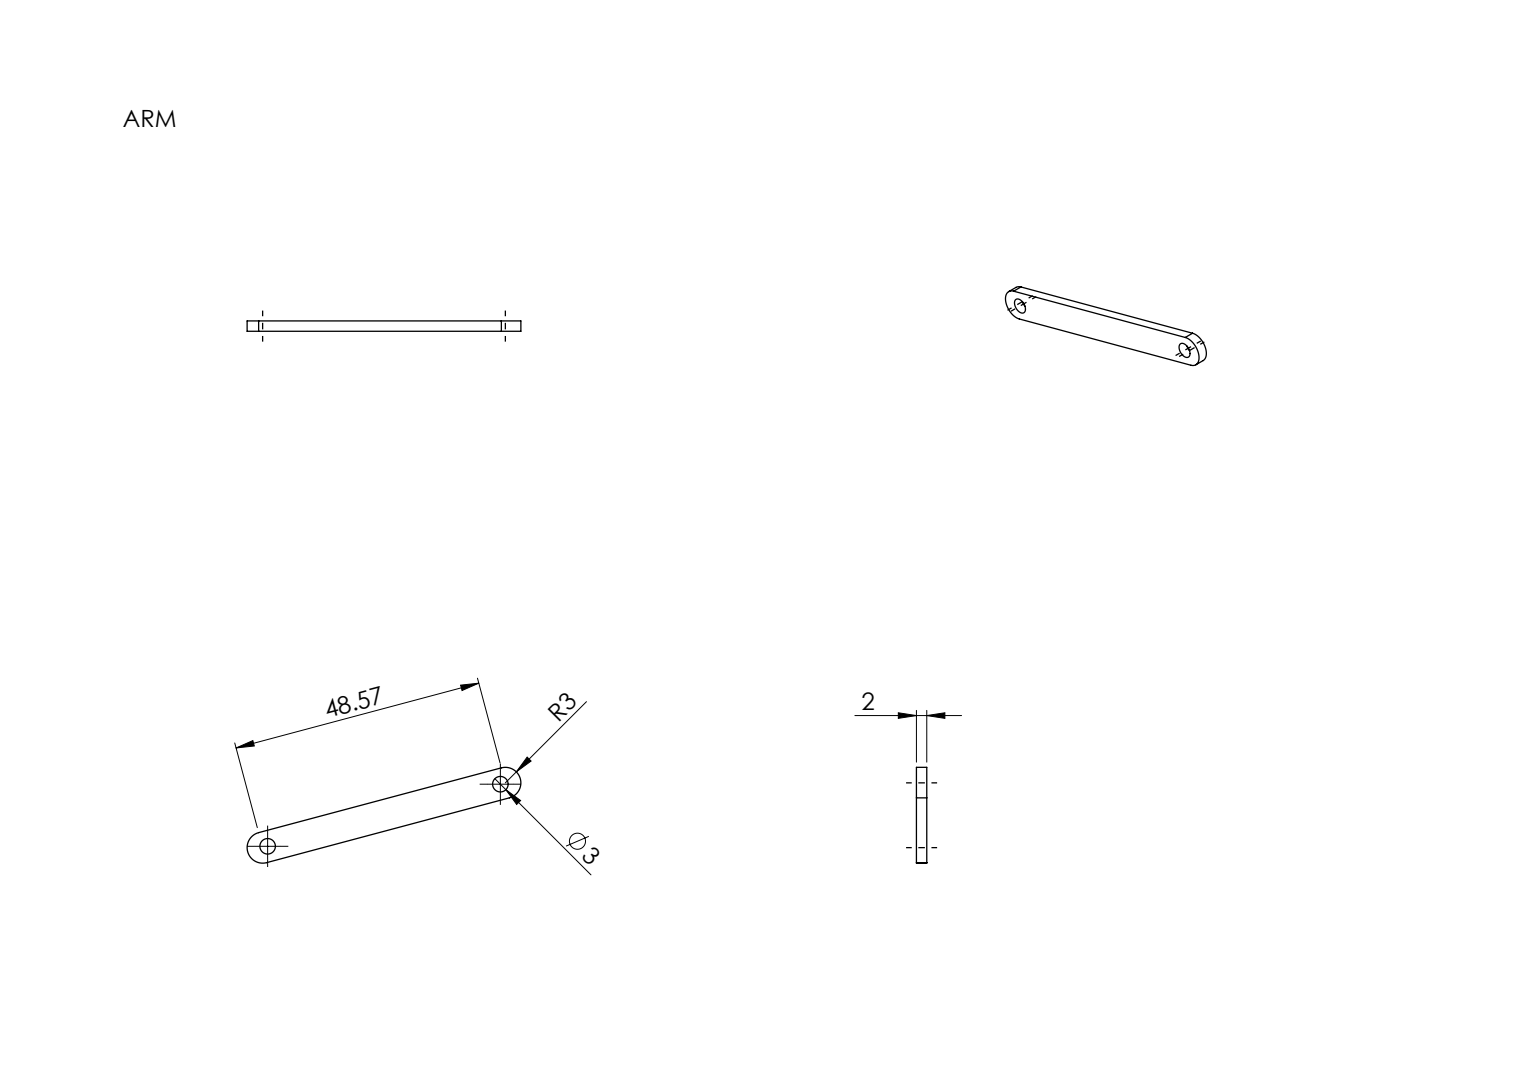
ISO-10303-21;
HEADER;
FILE_DESCRIPTION (('STEP AP214'),
    '1' );
FILE_NAME ('arm.step',
    '2026-10-04T07:56:41',
    ( '' ),
    ( '' ),
    'SwSTEP 2.0',
    'SolidWorks 2026',
    '' );
FILE_SCHEMA (( 'AUTOMOTIVE_DESIGN' ));
ENDSEC;

DATA;
#19=LINE ( 'NONE', #2774, #674 ) ;
#51=CIRCLE ( 'NONE', #1949, 3.000000000000000000 ) ;
#101=CARTESIAN_POINT ( 'NONE',  ( 46.73922289128223895, -17.64104216824340199, 4.500000000000000888 ) ) ;
#128=FACE_OUTER_BOUND ( 'NONE', #7423, .T. ) ;
#133=FACE_OUTER_BOUND ( 'NONE', #6862, .T. ) ;
#143=ORIENTED_EDGE ( 'NONE', *, *, #1238, .T. ) ;
#163=EDGE_LOOP ( 'NONE', ( #6818, #3032, #7905, #4249 ) ) ;
#171=FACE_OUTER_BOUND ( 'NONE', #565, .T. ) ;
#212=CARTESIAN_POINT ( 'NONE',  ( -0.9662349396012467340, -27.25766265056033433, 4.500000000000000888 ) ) ;
#225=SURFACE_STYLE_FILL_AREA ( #2174 ) ;
#261=CARTESIAN_POINT ( 'NONE',  ( 46.73922289128223895, -17.64104216824340199, 4.500000000000000888 ) ) ;
#270=DIRECTION ( 'NONE',  ( -0.000000000000000000, -0.000000000000000000, -1.000000000000000000 ) ) ;
#273=DIRECTION ( 'NONE',  ( 0.000000000000000000, 0.000000000000000000, 1.000000000000000000 ) ) ;
#277=ADVANCED_FACE ( 'NONE', ( #133 ), #3970, .F. ) ;
#318=LINE ( 'NONE', #2975, #6253 ) ;
#332=ORIENTED_EDGE ( 'NONE', *, *, #7144, .F. ) ;
#384=DIRECTION ( 'NONE',  ( -1.000000000000000000, 0.000000000000000000, 0.000000000000000000 ) ) ;
#386=AXIS2_PLACEMENT_3D ( 'NONE', #1428, #3953, #5087 ) ;
#402=CARTESIAN_POINT ( 'NONE',  ( 0.7729879516809982087, -29.89870481880373987, 4.500000000000000888 ) ) ;
#425=VERTEX_POINT ( 'NONE', #5144 ) ;
#426=CARTESIAN_POINT ( 'NONE',  ( 45.96623493960122886, -14.74233734943963192, 2.500000000000000888 ) ) ;
#468=( NAMED_UNIT ( * ) PLANE_ANGLE_UNIT ( ) SI_UNIT ( $, .RADIAN. ) );
#504=FACE_OUTER_BOUND ( 'NONE', #5035, .T. ) ;
#521=AXIS2_PLACEMENT_3D ( 'NONE', #5224, #627, #804 ) ;
#540=VERTEX_POINT ( 'NONE', #5837 ) ;
#565=EDGE_LOOP ( 'NONE', ( #768, #2129, #3059, #5475 ) ) ;
#577=VERTEX_POINT ( 'NONE', #7832 ) ;
#602=EDGE_CURVE ( 'NONE', #5645, #577, #5831, .T. ) ;
#627=DIRECTION ( 'NONE',  ( -0.000000000000000000, -0.000000000000000000, -1.000000000000000000 ) ) ;
#672=( GEOMETRIC_REPRESENTATION_CONTEXT ( 3 ) GLOBAL_UNCERTAINTY_ASSIGNED_CONTEXT ( ( #2169 ) ) GLOBAL_UNIT_ASSIGNED_CONTEXT ( ( #902, #4727, #5913 ) ) REPRESENTATION_CONTEXT ( 'NONE', 'WORKASPACE' ) );
#673=FACE_OUTER_BOUND ( 'NONE', #163, .T. ) ;
#674=VECTOR ( 'NONE', #2142, 1000.000000000000000 ) ;
#693=DIRECTION ( 'NONE',  ( 0.000000000000000000, 0.000000000000000000, 1.000000000000000000 ) ) ;
#705=ORIENTED_EDGE ( 'NONE', *, *, #1358, .T. ) ;
#729=CIRCLE ( 'NONE', #4630, 1.500000000000001998 ) ;
#768=ORIENTED_EDGE ( 'NONE', *, *, #6942, .T. ) ;
#772=( LENGTH_UNIT ( ) NAMED_UNIT ( * ) SI_UNIT ( .MILLI., .METRE. ) );
#777=EDGE_CURVE ( 'NONE', #3733, #7693, #19, .T. ) ;
#804=DIRECTION ( 'NONE',  ( -1.000000000000000000, 0.000000000000000000, 0.000000000000000000 ) ) ;
#805=CIRCLE ( 'NONE', #4298, 3.000000000000000000 ) ;
#816=EDGE_LOOP ( 'NONE', ( #5885, #8217, #3994, #3810 ) ) ;
#862=VECTOR ( 'NONE', #1618, 1000.000000000000227 ) ;
#902=( LENGTH_UNIT ( ) NAMED_UNIT ( * ) SI_UNIT ( .MILLI., .METRE. ) );
#937=EDGE_CURVE ( 'NONE', #8122, #5636, #7138, .T. ) ;
#944=VECTOR ( 'NONE', #2202, 1000.000000000000000 ) ;
#971=DIRECTION ( 'NONE',  ( -1.000000000000000000, 0.000000000000000000, 0.000000000000000000 ) ) ;
#980=CYLINDRICAL_SURFACE ( 'NONE', #1948, 1.499999999999994449 ) ;
#998=CIRCLE ( 'NONE', #3155, 1.500000000000001998 ) ;
#1037=ADVANCED_FACE ( 'NONE', ( #3889 ), #7135, .F. ) ;
#1053=DIRECTION ( 'NONE',  ( 0.000000000000000000, 0.000000000000000000, 1.000000000000000000 ) ) ;
#1078=CARTESIAN_POINT ( 'NONE',  ( 6.123233995736760366E-16, -27.00000000000000000, 4.500000000000000888 ) ) ;
#1102=FILL_AREA_STYLE ('',( #6916 ) ) ;
#1137=CARTESIAN_POINT ( 'NONE',  ( 45.96623493960122886, -14.74233734943963192, 4.500000000000000888 ) ) ;
#1238=EDGE_CURVE ( 'NONE', #3733, #5980, #6033, .T. ) ;
#1256=AXIS2_PLACEMENT_3D ( 'NONE', #1926, #3778, #2010 ) ;
#1265=( GEOMETRIC_REPRESENTATION_CONTEXT ( 3 ) GLOBAL_UNCERTAINTY_ASSIGNED_CONTEXT ( ( #3607 ) ) GLOBAL_UNIT_ASSIGNED_CONTEXT ( ( #7000, #468, #5646 ) ) REPRESENTATION_CONTEXT ( 'NONE', 'WORKASPACE' ) );
#1283=DIRECTION ( 'NONE',  ( 0.000000000000000000, 0.000000000000000000, 1.000000000000000000 ) ) ;
#1345=ORIENTED_EDGE ( 'NONE', *, *, #2125, .T. ) ;
#1358=EDGE_CURVE ( 'NONE', #8122, #577, #2207, .T. ) ;
#1392=PRODUCT_DEFINITION ( 'UNKNOWN', '', #2424, #5360 ) ;
#1394=PLANE ( 'NONE',  #6055 ) ;
#1402=DIRECTION ( 'NONE',  ( -1.000000000000000000, 0.000000000000000000, 0.000000000000000000 ) ) ;
#1428=CARTESIAN_POINT ( 'NONE',  ( 45.00000000000000000, -14.99999999999999467, 2.500000000000000888 ) ) ;
#1470=DIRECTION ( 'NONE',  ( -0.000000000000000000, -0.000000000000000000, -1.000000000000000000 ) ) ;
#1472=ORIENTED_EDGE ( 'NONE', *, *, #5256, .T. ) ;
#1493=( NAMED_UNIT ( * ) PLANE_ANGLE_UNIT ( ) SI_UNIT ( $, .RADIAN. ) );
#1536=VECTOR ( 'NONE', #1470, 1000.000000000000000 ) ;
#1541=CARTESIAN_POINT ( 'NONE',  ( 45.00000000000000000, -14.99999999999999467, 4.500000000000000888 ) ) ;
#1545=EDGE_CURVE ( 'NONE', #2326, #3416, #2265, .T. ) ;
#1594=VERTEX_POINT ( 'NONE', #6433 ) ;
#1605=CARTESIAN_POINT ( 'NONE',  ( 45.96623493960122886, -14.74233734943963192, 4.500000000000000888 ) ) ;
#1618=DIRECTION ( 'NONE',  ( 0.9662349396012460678, 0.2576626505603330508, -0.000000000000000000 ) ) ;
#1654=CARTESIAN_POINT ( 'NONE',  ( 45.19324698792023298, -11.84363253063589205, 4.500000000000000888 ) ) ;
#1674=AXIS2_PLACEMENT_3D ( 'NONE', #2882, #3591, #384 ) ;
#1728=VECTOR ( 'NONE', #6153, 1000.000000000000000 ) ;
#1731=ORIENTED_EDGE ( 'NONE', *, *, #2146, .T. ) ;
#1756=DIRECTION ( 'NONE',  ( 1.000000000000000000, 0.000000000000000000, 0.000000000000000000 ) ) ;
#1782=ORIENTED_EDGE ( 'NONE', *, *, #937, .T. ) ;
#1813=MECHANICAL_DESIGN_GEOMETRIC_PRESENTATION_REPRESENTATION('',(#6914),#1265);
#1818=CIRCLE ( 'NONE', #2086, 1.499999999999994449 ) ;
#1882=ORIENTED_EDGE ( 'NONE', *, *, #4850, .T. ) ;
#1926=CARTESIAN_POINT ( 'NONE',  ( -0.9662349396012467340, -27.25766265056033433, 2.500000000000000888 ) ) ;
#1933=SHAPE_REPRESENTATION ( 'arm', ( #2840 ), #5779 ) ;
#1946=EDGE_CURVE ( 'NONE', #1594, #540, #729, .T. ) ;
#1948=AXIS2_PLACEMENT_3D ( 'NONE', #4723, #2211, #6078 ) ;
#1949=AXIS2_PLACEMENT_3D ( 'NONE', #4301, #7678, #4461 ) ;
#1954=FACE_BOUND ( 'NONE', #3515, .T. ) ;
#1994=DIRECTION ( 'NONE',  ( 0.000000000000000000, 0.000000000000000000, 1.000000000000000000 ) ) ;
#2008=CARTESIAN_POINT ( 'NONE',  ( 45.00000000000000000, -14.99999999999999467, 4.500000000000000888 ) ) ;
#2010=DIRECTION ( 'NONE',  ( -1.000000000000000000, 0.000000000000000000, 0.000000000000000000 ) ) ;
#2016=CARTESIAN_POINT ( 'NONE',  ( 45.00000000000000000, -14.99999999999999467, 2.500000000000000888 ) ) ;
#2038=CARTESIAN_POINT ( 'NONE',  ( 6.123233995736760366E-16, -27.00000000000000000, 2.500000000000000888 ) ) ;
#2050=FILL_AREA_STYLE_COLOUR ( '', #3641 ) ;
#2077=CARTESIAN_POINT ( 'NONE',  ( 0.7729879516809982087, -29.89870481880373987, 4.500000000000000888 ) ) ;
#2086=AXIS2_PLACEMENT_3D ( 'NONE', #2008, #1283, #2469 ) ;
#2093=ORIENTED_EDGE ( 'NONE', *, *, #2146, .F. ) ;
#2111=ORIENTED_EDGE ( 'NONE', *, *, #6840, .F. ) ;
#2117=EDGE_CURVE ( 'NONE', #425, #6564, #6175, .T. ) ;
#2125=EDGE_CURVE ( 'NONE', #540, #2326, #318, .T. ) ;
#2129=ORIENTED_EDGE ( 'NONE', *, *, #7263, .F. ) ;
#2142=DIRECTION ( 'NONE',  ( -0.9662349396012451797, -0.2576626505603366590, -0.000000000000000000 ) ) ;
#2146=EDGE_CURVE ( 'NONE', #5636, #8122, #1818, .T. ) ;
#2149=CIRCLE ( 'NONE', #386, 1.499999999999994449 ) ;
#2169=UNCERTAINTY_MEASURE_WITH_UNIT (LENGTH_MEASURE( 1.000000000000000082E-05 ), #902, 'distance_accuracy_value', 'NONE');
#2174=FILL_AREA_STYLE ('',( #2050 ) ) ;
#2202=DIRECTION ( 'NONE',  ( -0.000000000000000000, -0.000000000000000000, -1.000000000000000000 ) ) ;
#2207=LINE ( 'NONE', #4719, #1728 ) ;
#2211=DIRECTION ( 'NONE',  ( -0.000000000000000000, -0.000000000000000000, -1.000000000000000000 ) ) ;
#2228=ORIENTED_EDGE ( 'NONE', *, *, #1545, .T. ) ;
#2246=FACE_OUTER_BOUND ( 'NONE', #816, .T. ) ;
#2255=ORIENTED_EDGE ( 'NONE', *, *, #937, .F. ) ;
#2265=CIRCLE ( 'NONE', #8315, 1.500000000000001998 ) ;
#2310=ORIENTED_EDGE ( 'NONE', *, *, #602, .F. ) ;
#2312=EDGE_LOOP ( 'NONE', ( #2228, #1882 ) ) ;
#2326=VERTEX_POINT ( 'NONE', #5199 ) ;
#2327=DIRECTION ( 'NONE',  ( 0.000000000000000000, 0.000000000000000000, 1.000000000000000000 ) ) ;
#2335=CARTESIAN_POINT ( 'NONE',  ( 0.7729879516809982087, -29.89870481880373987, 2.500000000000000888 ) ) ;
#2385=DIRECTION ( 'NONE',  ( 0.000000000000000000, 0.000000000000000000, 1.000000000000000000 ) ) ;
#2424=PRODUCT_DEFINITION_FORMATION_WITH_SPECIFIED_SOURCE ( 'ANY', '', #3664, .NOT_KNOWN. ) ;
#2469=DIRECTION ( 'NONE',  ( 1.000000000000000000, 0.000000000000000000, 0.000000000000000000 ) ) ;
#2475=CIRCLE ( 'NONE', #7188, 3.000000000000002665 ) ;
#2556=DIRECTION ( 'NONE',  ( -0.000000000000000000, -0.000000000000000000, -1.000000000000000000 ) ) ;
#2594=ADVANCED_FACE ( 'NONE', ( #4778 ), #2726, .T. ) ;
#2625=DIRECTION ( 'NONE',  ( 0.000000000000000000, 0.000000000000000000, 1.000000000000000000 ) ) ;
#2635=CLOSED_SHELL ( 'NONE', ( #1037, #4519, #4754, #4844, #6356, #7819, #6759, #2594, #7467, #277, #4433 ) ) ;
#2699=CARTESIAN_POINT ( 'NONE',  ( 46.49999999999999289, -14.99999999999999467, 2.500000000000000888 ) ) ;
#2715=CARTESIAN_POINT ( 'NONE',  ( 6.123233995736760366E-16, -27.00000000000000000, 4.500000000000000888 ) ) ;
#2726=CYLINDRICAL_SURFACE ( 'NONE', #4756, 3.000000000000000000 ) ;
#2729=EDGE_CURVE ( 'NONE', #7693, #2822, #6003, .T. ) ;
#2755=VECTOR ( 'NONE', #2556, 1000.000000000000000 ) ;
#2774=CARTESIAN_POINT ( 'NONE',  ( 44.22701204831900412, -12.10129518119625658, 4.500000000000000888 ) ) ;
#2804=ORIENTED_EDGE ( 'NONE', *, *, #602, .T. ) ;
#2812=ORIENTED_EDGE ( 'NONE', *, *, #5575, .F. ) ;
#2822=VERTEX_POINT ( 'NONE', #7439 ) ;
#2840=AXIS2_PLACEMENT_3D ( 'NONE', #8120, #5497, #1756 ) ;
#2877=LINE ( 'NONE', #6702, #6242 ) ;
#2882=CARTESIAN_POINT ( 'NONE',  ( -0.9662349396012467340, -27.25766265056033433, 4.500000000000000888 ) ) ;
#2963=DIRECTION ( 'NONE',  ( 0.000000000000000000, 0.000000000000000000, 1.000000000000000000 ) ) ;
#2975=CARTESIAN_POINT ( 'NONE',  ( -1.500000000000001332, -27.00000000000000000, 4.500000000000000888 ) ) ;
#2994=DIRECTION ( 'NONE',  ( 0.000000000000000000, 0.000000000000000000, 1.000000000000000000 ) ) ;
#3011=EDGE_CURVE ( 'NONE', #540, #1594, #998, .T. ) ;
#3032=ORIENTED_EDGE ( 'NONE', *, *, #4118, .T. ) ;
#3041=DIRECTION ( 'NONE',  ( -0.000000000000000000, -0.000000000000000000, -1.000000000000000000 ) ) ;
#3055=EDGE_LOOP ( 'NONE', ( #2111, #7565, #4948, #332, #7058 ) ) ;
#3059=ORIENTED_EDGE ( 'NONE', *, *, #2117, .F. ) ;
#3102=STYLED_ITEM ( 'NONE', ( #3979 ), #4379 ) ;
#3103=ORIENTED_EDGE ( 'NONE', *, *, #2125, .F. ) ;
#3104=CARTESIAN_POINT ( 'NONE',  ( 45.96623493960122886, -14.74233734943963192, 2.500000000000000888 ) ) ;
#3138=ORIENTED_EDGE ( 'NONE', *, *, #6646, .T. ) ;
#3155=AXIS2_PLACEMENT_3D ( 'NONE', #6255, #2385, #3645 ) ;
#3160=LINE ( 'NONE', #3790, #3546 ) ;
#3161=VECTOR ( 'NONE', #3731, 1000.000000000000114 ) ;
#3183=ORIENTED_EDGE ( 'NONE', *, *, #1946, .T. ) ;
#3295=AXIS2_PLACEMENT_3D ( 'NONE', #2016, #693, #6600 ) ;
#3296=COLOUR_RGB ( '', 0.66274510, 0.83137255, 0.94901961) ;
#3370=AXIS2_PLACEMENT_3D ( 'NONE', #1605, #4170, #971 ) ;
#3416=VERTEX_POINT ( 'NONE', #5319 ) ;
#3471=ORIENTED_EDGE ( 'NONE', *, *, #1545, .F. ) ;
#3515=EDGE_LOOP ( 'NONE', ( #4016, #3980 ) ) ;
#3521=DIRECTION ( 'NONE',  ( 1.000000000000000000, 0.000000000000000000, 0.000000000000000000 ) ) ;
#3525=ORIENTED_EDGE ( 'NONE', *, *, #2729, .F. ) ;
#3546=VECTOR ( 'NONE', #6361, 1000.000000000000000 ) ;
#3563=ORIENTED_EDGE ( 'NONE', *, *, #7749, .F. ) ;
#3581=ORIENTED_EDGE ( 'NONE', *, *, #7144, .T. ) ;
#3591=DIRECTION ( 'NONE',  ( 0.000000000000000000, 0.000000000000000000, 1.000000000000000000 ) ) ;
#3607=UNCERTAINTY_MEASURE_WITH_UNIT (LENGTH_MEASURE( 1.000000000000000082E-05 ), #7000, 'distance_accuracy_value', 'NONE');
#3641=COLOUR_RGB ( '', 0.66274510, 0.83137255, 0.94901961) ;
#3645=DIRECTION ( 'NONE',  ( 1.000000000000000000, 0.000000000000000000, 0.000000000000000000 ) ) ;
#3664=PRODUCT ( 'arm', 'arm', '', ( #5516 ) ) ;
#3731=DIRECTION ( 'NONE',  ( 0.9662349396012461789, 0.2576626505603324402, 0.000000000000000000 ) ) ;
#3733=VERTEX_POINT ( 'NONE', #1654 ) ;
#3734=FACE_BOUND ( 'NONE', #2312, .T. ) ;
#3773=EDGE_CURVE ( 'NONE', #5980, #2822, #2877, .T. ) ;
#3775=MECHANICAL_DESIGN_GEOMETRIC_PRESENTATION_REPRESENTATION('',(#3102),#672);
#3778=DIRECTION ( 'NONE',  ( 0.000000000000000000, 0.000000000000000000, 1.000000000000000000 ) ) ;
#3790=CARTESIAN_POINT ( 'NONE',  ( -3.966234939601246623, -27.25766265056033433, 4.500000000000000888 ) ) ;
#3810=ORIENTED_EDGE ( 'NONE', *, *, #7263, .T. ) ;
#3876=AXIS2_PLACEMENT_3D ( 'NONE', #7856, #7176, #1402 ) ;
#3889=FACE_OUTER_BOUND ( 'NONE', #7158, .T. ) ;
#3952=VERTEX_POINT ( 'NONE', #6989 ) ;
#3953=DIRECTION ( 'NONE',  ( 0.000000000000000000, 0.000000000000000000, 1.000000000000000000 ) ) ;
#3970=CYLINDRICAL_SURFACE ( 'NONE', #4962, 1.500000000000001998 ) ;
#3979=PRESENTATION_STYLE_ASSIGNMENT (( #5325 ) ) ;
#3980=ORIENTED_EDGE ( 'NONE', *, *, #1946, .F. ) ;
#3982=DIRECTION ( 'NONE',  ( -0.000000000000000000, -0.000000000000000000, -1.000000000000000000 ) ) ;
#3994=ORIENTED_EDGE ( 'NONE', *, *, #5256, .F. ) ;
#4016=ORIENTED_EDGE ( 'NONE', *, *, #3011, .F. ) ;
#4118=EDGE_CURVE ( 'NONE', #5910, #8028, #3160, .T. ) ;
#4140=PLANE ( 'NONE',  #4751 ) ;
#4156=CARTESIAN_POINT ( 'NONE',  ( -3.966234939601246623, -27.25766265056033433, 4.500000000000000888 ) ) ;
#4170=DIRECTION ( 'NONE',  ( -0.000000000000000000, -0.000000000000000000, -1.000000000000000000 ) ) ;
#4183=EDGE_LOOP ( 'NONE', ( #5342, #6201, #5935, #3581 ) ) ;
#4189=EDGE_CURVE ( 'NONE', #425, #6172, #7925, .T. ) ;
#4218=CIRCLE ( 'NONE', #1674, 3.000000000000000000 ) ;
#4220=CARTESIAN_POINT ( 'NONE',  ( -0.7729879516809968765, -24.10129518119626013, 4.500000000000000888 ) ) ;
#4249=ORIENTED_EDGE ( 'NONE', *, *, #4189, .F. ) ;
#4298=AXIS2_PLACEMENT_3D ( 'NONE', #212, #2327, #6697 ) ;
#4301=CARTESIAN_POINT ( 'NONE',  ( -0.9662349396012467340, -27.25766265056033433, 2.500000000000000888 ) ) ;
#4379=ADVANCED_BREP_SHAPE_REPRESENTATION ( '', ( #7177, #2840 ), #5779 ) ;
#4417=SURFACE_STYLE_FILL_AREA ( #1102 ) ;
#4433=ADVANCED_FACE ( 'NONE', ( #8066 ), #980, .F. ) ;
#4461=DIRECTION ( 'NONE',  ( -1.000000000000000000, 0.000000000000000000, 0.000000000000000000 ) ) ;
#4474=ORIENTED_EDGE ( 'NONE', *, *, #2117, .T. ) ;
#4490=VECTOR ( 'NONE', #270, 1000.000000000000000 ) ;
#4519=ADVANCED_FACE ( 'NONE', ( #504 ), #5725, .F. ) ;
#4561=AXIS2_PLACEMENT_3D ( 'NONE', #1541, #273, #3521 ) ;
#4630=AXIS2_PLACEMENT_3D ( 'NONE', #1078, #8041, #5542 ) ;
#4631=CARTESIAN_POINT ( 'NONE',  ( 45.96623493960122886, -14.74233734943963192, 4.500000000000000888 ) ) ;
#4632=DIRECTION ( 'NONE',  ( -0.2576626505603331063, 0.9662349396012461789, 0.000000000000000000 ) ) ;
#4646=SURFACE_SIDE_STYLE ('',( #225 ) ) ;
#4688=AXIS2_PLACEMENT_3D ( 'NONE', #1137, #1053, #4929 ) ;
#4719=CARTESIAN_POINT ( 'NONE',  ( 43.50000000000000711, -14.99999999999999467, 4.500000000000000888 ) ) ;
#4723=CARTESIAN_POINT ( 'NONE',  ( 45.00000000000000000, -14.99999999999999467, 4.500000000000000888 ) ) ;
#4727=( NAMED_UNIT ( * ) PLANE_ANGLE_UNIT ( ) SI_UNIT ( $, .RADIAN. ) );
#4751=AXIS2_PLACEMENT_3D ( 'NONE', #4220, #4771, #6120 ) ;
#4754=ADVANCED_FACE ( 'NONE', ( #673 ), #7126, .T. ) ;
#4756=AXIS2_PLACEMENT_3D ( 'NONE', #7910, #3982, #5917 ) ;
#4771=DIRECTION ( 'NONE',  ( 0.2576626505603332173, -0.9662349396012460678, 0.000000000000000000 ) ) ;
#4778=FACE_OUTER_BOUND ( 'NONE', #4183, .T. ) ;
#4801=CYLINDRICAL_SURFACE ( 'NONE', #3370, 3.000000000000002665 ) ;
#4844=ADVANCED_FACE ( 'NONE', ( #1954, #128, #5855 ), #5269, .T. ) ;
#4850=EDGE_CURVE ( 'NONE', #3416, #2326, #6986, .T. ) ;
#4892=CIRCLE ( 'NONE', #1256, 3.000000000000000000 ) ;
#4894=CARTESIAN_POINT ( 'NONE',  ( 6.123233995736760366E-16, -27.00000000000000000, 2.500000000000000888 ) ) ;
#4918=FACE_OUTER_BOUND ( 'NONE', #3055, .T. ) ;
#4929=DIRECTION ( 'NONE',  ( 1.000000000000000000, 0.000000000000000000, 0.000000000000000000 ) ) ;
#4948=ORIENTED_EDGE ( 'NONE', *, *, #6418, .F. ) ;
#4951=FACE_BOUND ( 'NONE', #5931, .T. ) ;
#4962=AXIS2_PLACEMENT_3D ( 'NONE', #2715, #5273, #7767 ) ;
#4964=ORIENTED_EDGE ( 'NONE', *, *, #7749, .T. ) ;
#4977=SURFACE_STYLE_USAGE ( .BOTH. , #8186 ) ;
#4994=CARTESIAN_POINT ( 'NONE',  ( -0.1932469879202498297, -30.15636746936407064, 2.500000000000000888 ) ) ;
#5015=DIRECTION ( 'NONE',  ( -1.000000000000000000, 0.000000000000000000, 0.000000000000000000 ) ) ;
#5035=EDGE_LOOP ( 'NONE', ( #7861, #3138, #3471, #3103 ) ) ;
#5074=EDGE_LOOP ( 'NONE', ( #2255, #2093 ) ) ;
#5087=DIRECTION ( 'NONE',  ( 1.000000000000000000, 0.000000000000000000, 0.000000000000000000 ) ) ;
#5144=CARTESIAN_POINT ( 'NONE',  ( -0.1932469879202498297, -30.15636746936407064, 4.500000000000000888 ) ) ;
#5185=DIRECTION ( 'NONE',  ( 1.000000000000000000, 0.000000000000000000, -0.000000000000000000 ) ) ;
#5199=CARTESIAN_POINT ( 'NONE',  ( -1.500000000000001332, -27.00000000000000000, 2.500000000000000888 ) ) ;
#5224=CARTESIAN_POINT ( 'NONE',  ( -0.9662349396012467340, -27.25766265056033433, 4.500000000000000888 ) ) ;
#5256=EDGE_CURVE ( 'NONE', #6564, #3733, #6710, .T. ) ;
#5269=PLANE ( 'NONE',  #5908 ) ;
#5273=DIRECTION ( 'NONE',  ( -0.000000000000000000, -0.000000000000000000, -1.000000000000000000 ) ) ;
#5304=ORIENTED_EDGE ( 'NONE', *, *, #5575, .T. ) ;
#5319=CARTESIAN_POINT ( 'NONE',  ( 1.500000000000002665, -27.00000000000000000, 2.500000000000000888 ) ) ;
#5325=SURFACE_STYLE_USAGE ( .BOTH. , #4646 ) ;
#5342=ORIENTED_EDGE ( 'NONE', *, *, #4118, .F. ) ;
#5360=PRODUCT_DEFINITION_CONTEXT ( 'detailed design', #6318, 'design' ) ;
#5367=CARTESIAN_POINT ( 'NONE',  ( -1.739222891282244055, -24.35895783175659446, 4.500000000000000888 ) ) ;
#5475=ORIENTED_EDGE ( 'NONE', *, *, #4189, .T. ) ;
#5479=CARTESIAN_POINT ( 'NONE',  ( -1.739222891282244055, -24.35895783175659446, 4.500000000000000888 ) ) ;
#5497=DIRECTION ( 'NONE',  ( 0.000000000000000000, 0.000000000000000000, 1.000000000000000000 ) ) ;
#5516=PRODUCT_CONTEXT ( 'NONE', #7773, 'mechanical' ) ;
#5542=DIRECTION ( 'NONE',  ( 1.000000000000000000, 0.000000000000000000, 0.000000000000000000 ) ) ;
#5566=PRESENTATION_STYLE_ASSIGNMENT (( #4977 ) ) ;
#5575=EDGE_CURVE ( 'NONE', #577, #5645, #2149, .T. ) ;
#5620=PLANE ( 'NONE',  #6639 ) ;
#5636=VERTEX_POINT ( 'NONE', #7667 ) ;
#5639=ORIENTED_EDGE ( 'NONE', *, *, #7587, .T. ) ;
#5645=VERTEX_POINT ( 'NONE', #2699 ) ;
#5646=( NAMED_UNIT ( * ) SI_UNIT ( $, .STERADIAN. ) SOLID_ANGLE_UNIT ( ) );
#5657=EDGE_LOOP ( 'NONE', ( #3563, #1731, #705, #2310 ) ) ;
#5701=LINE ( 'NONE', #8282, #2755 ) ;
#5725=CYLINDRICAL_SURFACE ( 'NONE', #6587, 1.500000000000001998 ) ;
#5779=( GEOMETRIC_REPRESENTATION_CONTEXT ( 3 ) GLOBAL_UNCERTAINTY_ASSIGNED_CONTEXT ( ( #6036 ) ) GLOBAL_UNIT_ASSIGNED_CONTEXT ( ( #772, #1493, #6712 ) ) REPRESENTATION_CONTEXT ( 'NONE', 'WORKASPACE' ) );
#5822=EDGE_LOOP ( 'NONE', ( #6359, #3525, #6764, #143 ) ) ;
#5831=CIRCLE ( 'NONE', #3295, 1.499999999999994449 ) ;
#5837=CARTESIAN_POINT ( 'NONE',  ( -1.500000000000001332, -27.00000000000000000, 4.500000000000000888 ) ) ;
#5855=FACE_BOUND ( 'NONE', #5074, .T. ) ;
#5885=ORIENTED_EDGE ( 'NONE', *, *, #6840, .T. ) ;
#5908=AXIS2_PLACEMENT_3D ( 'NONE', #4631, #2625, #5185 ) ;
#5910=VERTEX_POINT ( 'NONE', #4156 ) ;
#5913=( NAMED_UNIT ( * ) SI_UNIT ( $, .STERADIAN. ) SOLID_ANGLE_UNIT ( ) );
#5917=DIRECTION ( 'NONE',  ( -1.000000000000000000, 0.000000000000000000, 0.000000000000000000 ) ) ;
#5931=EDGE_LOOP ( 'NONE', ( #5304, #2804 ) ) ;
#5932=CARTESIAN_POINT ( 'NONE',  ( 45.19324698792023298, -11.84363253063589205, 2.500000000000000888 ) ) ;
#5935=ORIENTED_EDGE ( 'NONE', *, *, #2729, .T. ) ;
#5980=VERTEX_POINT ( 'NONE', #5932 ) ;
#5989=CARTESIAN_POINT ( 'NONE',  ( 46.49999999999999289, -14.99999999999999467, 4.500000000000000888 ) ) ;
#6003=LINE ( 'NONE', #5367, #4490 ) ;
#6033=LINE ( 'NONE', #6701, #6157 ) ;
#6036=UNCERTAINTY_MEASURE_WITH_UNIT (LENGTH_MEASURE( 1.000000000000000082E-05 ), #772, 'distance_accuracy_value', 'NONE');
#6055=AXIS2_PLACEMENT_3D ( 'NONE', #2077, #4632, #6492 ) ;
#6078=DIRECTION ( 'NONE',  ( -1.000000000000000000, 0.000000000000000000, 0.000000000000000000 ) ) ;
#6120=DIRECTION ( 'NONE',  ( 0.9662349396012460678, 0.2576626505603332173, 0.000000000000000000 ) ) ;
#6153=DIRECTION ( 'NONE',  ( -0.000000000000000000, -0.000000000000000000, -1.000000000000000000 ) ) ;
#6157=VECTOR ( 'NONE', #7901, 1000.000000000000000 ) ;
#6172=VERTEX_POINT ( 'NONE', #4994 ) ;
#6175=LINE ( 'NONE', #402, #3161 ) ;
#6201=ORIENTED_EDGE ( 'NONE', *, *, #6889, .F. ) ;
#6242=VECTOR ( 'NONE', #7382, 1000.000000000000114 ) ;
#6253=VECTOR ( 'NONE', #8123, 1000.000000000000000 ) ;
#6255=CARTESIAN_POINT ( 'NONE',  ( 6.123233995736760366E-16, -27.00000000000000000, 4.500000000000000888 ) ) ;
#6304=DIRECTION ( 'NONE',  ( 0.000000000000000000, 0.000000000000000000, 1.000000000000000000 ) ) ;
#6318=APPLICATION_CONTEXT ( 'automotive_design' ) ;
#6330=CARTESIAN_POINT ( 'NONE',  ( 6.123233995736760366E-16, -27.00000000000000000, 4.500000000000000888 ) ) ;
#6356=ADVANCED_FACE ( 'NONE', ( #4918, #3734, #4951 ), #5620, .F. ) ;
#6359=ORIENTED_EDGE ( 'NONE', *, *, #3773, .T. ) ;
#6361=DIRECTION ( 'NONE',  ( -0.000000000000000000, -0.000000000000000000, -1.000000000000000000 ) ) ;
#6362=PRODUCT_DEFINITION_SHAPE ( 'NONE', 'NONE',  #1392 ) ;
#6418=EDGE_CURVE ( 'NONE', #8028, #6172, #4892, .T. ) ;
#6424=SHAPE_DEFINITION_REPRESENTATION ( #6362, #1933 ) ;
#6433=CARTESIAN_POINT ( 'NONE',  ( 1.500000000000002665, -27.00000000000000000, 4.500000000000000888 ) ) ;
#6492=DIRECTION ( 'NONE',  ( -0.9662349396012460678, -0.2576626505603330508, 0.000000000000000000 ) ) ;
#6551=DIRECTION ( 'NONE',  ( 1.000000000000000000, 0.000000000000000000, 0.000000000000000000 ) ) ;
#6564=VERTEX_POINT ( 'NONE', #101 ) ;
#6587=AXIS2_PLACEMENT_3D ( 'NONE', #6330, #3041, #5015 ) ;
#6600=DIRECTION ( 'NONE',  ( 1.000000000000000000, 0.000000000000000000, 0.000000000000000000 ) ) ;
#6639=AXIS2_PLACEMENT_3D ( 'NONE', #3104, #6304, #7529 ) ;
#6646=EDGE_CURVE ( 'NONE', #1594, #3416, #5701, .T. ) ;
#6697=DIRECTION ( 'NONE',  ( -1.000000000000000000, 0.000000000000000000, 0.000000000000000000 ) ) ;
#6701=CARTESIAN_POINT ( 'NONE',  ( 45.19324698792023298, -11.84363253063589205, 4.500000000000000888 ) ) ;
#6702=CARTESIAN_POINT ( 'NONE',  ( -0.7729879516809968765, -24.10129518119626013, 2.500000000000000888 ) ) ;
#6710=CIRCLE ( 'NONE', #4688, 3.000000000000002665 ) ;
#6712=( NAMED_UNIT ( * ) SI_UNIT ( $, .STERADIAN. ) SOLID_ANGLE_UNIT ( ) );
#6759=ADVANCED_FACE ( 'NONE', ( #8068 ), #4140, .F. ) ;
#6764=ORIENTED_EDGE ( 'NONE', *, *, #777, .F. ) ;
#6793=LINE ( 'NONE', #2335, #862 ) ;
#6806=ORIENTED_EDGE ( 'NONE', *, *, #777, .T. ) ;
#6818=ORIENTED_EDGE ( 'NONE', *, *, #7587, .F. ) ;
#6840=EDGE_CURVE ( 'NONE', #3952, #5980, #2475, .T. ) ;
#6849=ORIENTED_EDGE ( 'NONE', *, *, #4850, .F. ) ;
#6862=EDGE_LOOP ( 'NONE', ( #8336, #3183, #1345, #6849 ) ) ;
#6889=EDGE_CURVE ( 'NONE', #7693, #5910, #4218, .T. ) ;
#6914=STYLED_ITEM ( 'NONE', ( #5566 ), #7177 ) ;
#6916=FILL_AREA_STYLE_COLOUR ( '', #3296 ) ;
#6942=EDGE_CURVE ( 'NONE', #6172, #3952, #6793, .T. ) ;
#6986=CIRCLE ( 'NONE', #8077, 1.500000000000001998 ) ;
#6989=CARTESIAN_POINT ( 'NONE',  ( 46.73922289128223895, -17.64104216824340199, 2.500000000000000888 ) ) ;
#7000=( LENGTH_UNIT ( ) NAMED_UNIT ( * ) SI_UNIT ( .MILLI., .METRE. ) );
#7058=ORIENTED_EDGE ( 'NONE', *, *, #3773, .F. ) ;
#7126=CYLINDRICAL_SURFACE ( 'NONE', #521, 3.000000000000000000 ) ;
#7135=CYLINDRICAL_SURFACE ( 'NONE', #3876, 1.499999999999994449 ) ;
#7138=CIRCLE ( 'NONE', #4561, 1.499999999999994449 ) ;
#7144=EDGE_CURVE ( 'NONE', #2822, #8028, #51, .T. ) ;
#7158=EDGE_LOOP ( 'NONE', ( #1782, #4964, #2812, #7908 ) ) ;
#7170=LINE ( 'NONE', #261, #7401 ) ;
#7176=DIRECTION ( 'NONE',  ( -0.000000000000000000, -0.000000000000000000, -1.000000000000000000 ) ) ;
#7177=MANIFOLD_SOLID_BREP ( 'Boss-Extrude1', #2635 ) ;
#7188=AXIS2_PLACEMENT_3D ( 'NONE', #426, #2963, #6551 ) ;
#7228=SHAPE_REPRESENTATION_RELATIONSHIP ( 'NONE' , 'NONE' ,  #1933, #4379 ) ;
#7263=EDGE_CURVE ( 'NONE', #6564, #3952, #7170, .T. ) ;
#7382=DIRECTION ( 'NONE',  ( -0.9662349396012460678, -0.2576626505603332173, 0.000000000000000000 ) ) ;
#7401=VECTOR ( 'NONE', #7808, 1000.000000000000000 ) ;
#7423=EDGE_LOOP ( 'NONE', ( #4474, #1472, #6806, #7649, #5639 ) ) ;
#7439=CARTESIAN_POINT ( 'NONE',  ( -1.739222891282244055, -24.35895783175659446, 2.500000000000000888 ) ) ;
#7467=ADVANCED_FACE ( 'NONE', ( #171 ), #1394, .F. ) ;
#7529=DIRECTION ( 'NONE',  ( 1.000000000000000000, 0.000000000000000000, -0.000000000000000000 ) ) ;
#7565=ORIENTED_EDGE ( 'NONE', *, *, #6942, .F. ) ;
#7587=EDGE_CURVE ( 'NONE', #5910, #425, #805, .T. ) ;
#7649=ORIENTED_EDGE ( 'NONE', *, *, #6889, .T. ) ;
#7667=CARTESIAN_POINT ( 'NONE',  ( 46.49999999999999289, -14.99999999999999467, 4.500000000000000888 ) ) ;
#7678=DIRECTION ( 'NONE',  ( 0.000000000000000000, 0.000000000000000000, 1.000000000000000000 ) ) ;
#7693=VERTEX_POINT ( 'NONE', #5479 ) ;
#7697=CARTESIAN_POINT ( 'NONE',  ( -3.966234939601246623, -27.25766265056033433, 2.500000000000000888 ) ) ;
#7749=EDGE_CURVE ( 'NONE', #5636, #5645, #7976, .T. ) ;
#7767=DIRECTION ( 'NONE',  ( -1.000000000000000000, 0.000000000000000000, 0.000000000000000000 ) ) ;
#7773=APPLICATION_CONTEXT ( 'automotive_design' ) ;
#7808=DIRECTION ( 'NONE',  ( -0.000000000000000000, -0.000000000000000000, -1.000000000000000000 ) ) ;
#7819=ADVANCED_FACE ( 'NONE', ( #2246 ), #4801, .T. ) ;
#7832=CARTESIAN_POINT ( 'NONE',  ( 43.50000000000000711, -14.99999999999999467, 2.500000000000000888 ) ) ;
#7850=DIRECTION ( 'NONE',  ( 1.000000000000000000, 0.000000000000000000, 0.000000000000000000 ) ) ;
#7856=CARTESIAN_POINT ( 'NONE',  ( 45.00000000000000000, -14.99999999999999467, 4.500000000000000888 ) ) ;
#7861=ORIENTED_EDGE ( 'NONE', *, *, #3011, .T. ) ;
#7901=DIRECTION ( 'NONE',  ( -0.000000000000000000, -0.000000000000000000, -1.000000000000000000 ) ) ;
#7905=ORIENTED_EDGE ( 'NONE', *, *, #6418, .T. ) ;
#7908=ORIENTED_EDGE ( 'NONE', *, *, #1358, .F. ) ;
#7910=CARTESIAN_POINT ( 'NONE',  ( -0.9662349396012467340, -27.25766265056033433, 4.500000000000000888 ) ) ;
#7925=LINE ( 'NONE', #7965, #1536 ) ;
#7965=CARTESIAN_POINT ( 'NONE',  ( -0.1932469879202498297, -30.15636746936407064, 4.500000000000000888 ) ) ;
#7976=LINE ( 'NONE', #5989, #944 ) ;
#7994=CARTESIAN_POINT ( 'NONE',  ( 43.50000000000000711, -14.99999999999999467, 4.500000000000000888 ) ) ;
#8028=VERTEX_POINT ( 'NONE', #7697 ) ;
#8041=DIRECTION ( 'NONE',  ( 0.000000000000000000, 0.000000000000000000, 1.000000000000000000 ) ) ;
#8066=FACE_OUTER_BOUND ( 'NONE', #5657, .T. ) ;
#8068=FACE_OUTER_BOUND ( 'NONE', #5822, .T. ) ;
#8077=AXIS2_PLACEMENT_3D ( 'NONE', #2038, #1994, #7850 ) ;
#8120=CARTESIAN_POINT ( 'NONE',  ( 0.000000000000000000, 0.000000000000000000, 0.000000000000000000 ) ) ;
#8122=VERTEX_POINT ( 'NONE', #7994 ) ;
#8123=DIRECTION ( 'NONE',  ( -0.000000000000000000, -0.000000000000000000, -1.000000000000000000 ) ) ;
#8181=DIRECTION ( 'NONE',  ( 1.000000000000000000, 0.000000000000000000, 0.000000000000000000 ) ) ;
#8186=SURFACE_SIDE_STYLE ('',( #4417 ) ) ;
#8217=ORIENTED_EDGE ( 'NONE', *, *, #1238, .F. ) ;
#8282=CARTESIAN_POINT ( 'NONE',  ( 1.500000000000002665, -27.00000000000000000, 4.500000000000000888 ) ) ;
#8315=AXIS2_PLACEMENT_3D ( 'NONE', #4894, #2994, #8181 ) ;
#8336=ORIENTED_EDGE ( 'NONE', *, *, #6646, .F. ) ;
ENDSEC;
END-ISO-10303-21;
